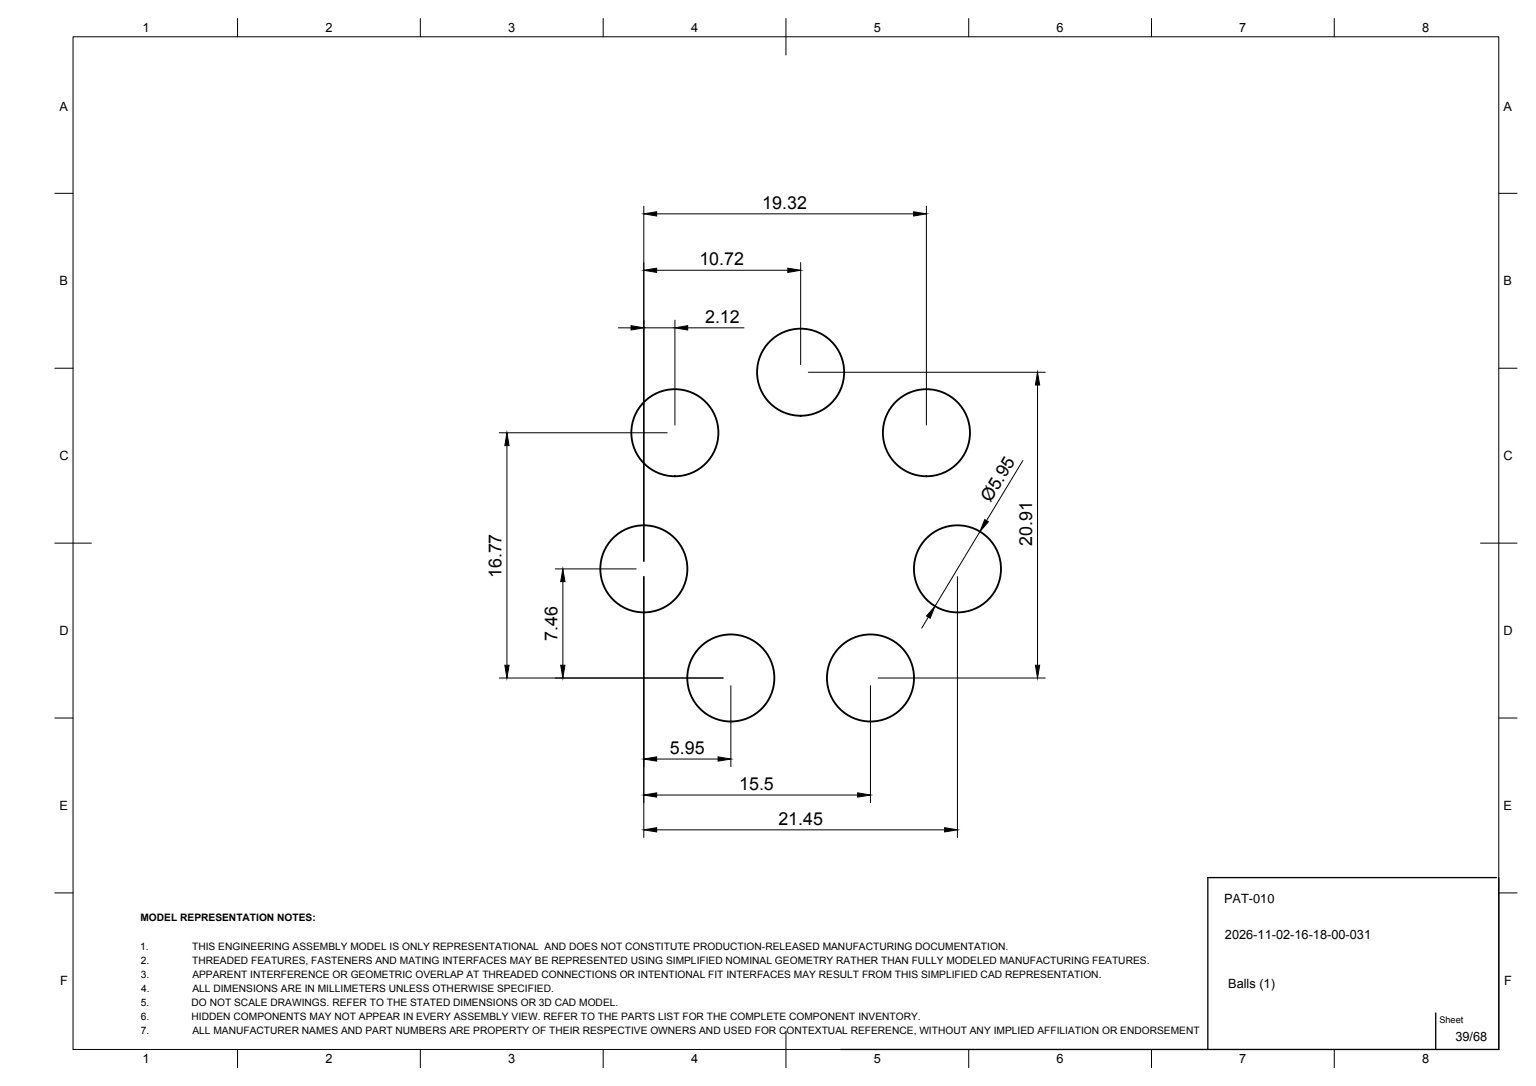
ISO-10303-21;
HEADER;
/* Generated by software containing ST-Developer
 * from STEP Tools, Inc. (www.steptools.com) 
 */

FILE_DESCRIPTION(
/* description */ ('Belt conveyor head drive unit'),
/* implementation_level */ '2;1');

FILE_NAME(
/* name */ 'Balls (1).step',
/* time_stamp */ '2026-10-28T03:26:19-07:00',
/* author */ (''),
/* organization */ (''),
/* preprocessor_version */ 'ST-DEVELOPER v20.2',
/* originating_system */ 'Autodesk Translation Framework v15.17.0.0',
/* authorisation */ '');

FILE_SCHEMA (('AUTOMOTIVE_DESIGN { 1 0 10303 214 3 1 1 }'));
ENDSEC;

DATA;
#10=MECHANICAL_DESIGN_GEOMETRIC_PRESENTATION_REPRESENTATION('',(#890,#891,#892,#893,#894,#895,#896),#27069);
#661=SPHERICAL_SURFACE('',#15395,0.29765);
#662=SPHERICAL_SURFACE('',#15397,0.29765);
#663=SPHERICAL_SURFACE('',#15399,0.29765);
#664=SPHERICAL_SURFACE('',#15401,0.29765);
#665=SPHERICAL_SURFACE('',#15403,0.29765);
#666=SPHERICAL_SURFACE('',#15405,0.29765);
#667=SPHERICAL_SURFACE('',#15407,0.29765);
#744=SHAPE_REPRESENTATION_RELATIONSHIP('SRR','None',#27390,#813);
#813=ADVANCED_BREP_SHAPE_REPRESENTATION('',(#974,#975,#976,#977,#978,#979,
#980),#27032);
#890=STYLED_ITEM('',(#27797),#974);
#891=STYLED_ITEM('',(#27797),#975);
#892=STYLED_ITEM('',(#27797),#976);
#893=STYLED_ITEM('',(#27797),#977);
#894=STYLED_ITEM('',(#27797),#978);
#895=STYLED_ITEM('',(#27797),#979);
#896=STYLED_ITEM('',(#27797),#980);
#974=MANIFOLD_SOLID_BREP('Body1',#13756);
#975=MANIFOLD_SOLID_BREP('Body2',#13757);
#976=MANIFOLD_SOLID_BREP('Body3',#13758);
#977=MANIFOLD_SOLID_BREP('Body4',#13759);
#978=MANIFOLD_SOLID_BREP('Body5',#13760);
#979=MANIFOLD_SOLID_BREP('Body6',#13761);
#980=MANIFOLD_SOLID_BREP('Body7',#13762);
#2021=FACE_OUTER_BOUND('',#2975,.T.);
#2022=FACE_OUTER_BOUND('',#2976,.T.);
#2023=FACE_OUTER_BOUND('',#2977,.T.);
#2024=FACE_OUTER_BOUND('',#2978,.T.);
#2025=FACE_OUTER_BOUND('',#2979,.T.);
#2026=FACE_OUTER_BOUND('',#2980,.T.);
#2027=FACE_OUTER_BOUND('',#2981,.T.);
#2975=EDGE_LOOP('',(#10618,#10619));
#2976=EDGE_LOOP('',(#10620,#10621));
#2977=EDGE_LOOP('',(#10622,#10623));
#2978=EDGE_LOOP('',(#10624,#10625));
#2979=EDGE_LOOP('',(#10626,#10627));
#2980=EDGE_LOOP('',(#10628,#10629));
#2981=EDGE_LOOP('',(#10630,#10631));
#5482=CIRCLE('',#15396,0.29765);
#5483=CIRCLE('',#15398,0.29765);
#5484=CIRCLE('',#15400,0.29765);
#5485=CIRCLE('',#15402,0.29765);
#5486=CIRCLE('',#15404,0.29765);
#5487=CIRCLE('',#15406,0.29765);
#5488=CIRCLE('',#15408,0.29765);
#6513=VERTEX_POINT('',#23132);
#6514=VERTEX_POINT('',#23133);
#6515=VERTEX_POINT('',#23136);
#6516=VERTEX_POINT('',#23137);
#6517=VERTEX_POINT('',#23140);
#6518=VERTEX_POINT('',#23141);
#6519=VERTEX_POINT('',#23144);
#6520=VERTEX_POINT('',#23145);
#6521=VERTEX_POINT('',#23148);
#6522=VERTEX_POINT('',#23149);
#6523=VERTEX_POINT('',#23152);
#6524=VERTEX_POINT('',#23153);
#6525=VERTEX_POINT('',#23156);
#6526=VERTEX_POINT('',#23157);
#8001=EDGE_CURVE('',#6513,#6514,#5482,.T.);
#8002=EDGE_CURVE('',#6515,#6516,#5483,.T.);
#8003=EDGE_CURVE('',#6517,#6518,#5484,.T.);
#8004=EDGE_CURVE('',#6519,#6520,#5485,.T.);
#8005=EDGE_CURVE('',#6521,#6522,#5486,.T.);
#8006=EDGE_CURVE('',#6523,#6524,#5487,.T.);
#8007=EDGE_CURVE('',#6525,#6526,#5488,.T.);
#10618=ORIENTED_EDGE('',*,*,#8001,.T.);
#10619=ORIENTED_EDGE('',*,*,#8001,.F.);
#10620=ORIENTED_EDGE('',*,*,#8002,.T.);
#10621=ORIENTED_EDGE('',*,*,#8002,.F.);
#10622=ORIENTED_EDGE('',*,*,#8003,.T.);
#10623=ORIENTED_EDGE('',*,*,#8003,.F.);
#10624=ORIENTED_EDGE('',*,*,#8004,.T.);
#10625=ORIENTED_EDGE('',*,*,#8004,.F.);
#10626=ORIENTED_EDGE('',*,*,#8005,.T.);
#10627=ORIENTED_EDGE('',*,*,#8005,.F.);
#10628=ORIENTED_EDGE('',*,*,#8006,.T.);
#10629=ORIENTED_EDGE('',*,*,#8006,.F.);
#10630=ORIENTED_EDGE('',*,*,#8007,.T.);
#10631=ORIENTED_EDGE('',*,*,#8007,.F.);
#13300=ADVANCED_FACE('',(#2021),#661,.T.);
#13301=ADVANCED_FACE('',(#2022),#662,.T.);
#13302=ADVANCED_FACE('',(#2023),#663,.T.);
#13303=ADVANCED_FACE('',(#2024),#664,.T.);
#13304=ADVANCED_FACE('',(#2025),#665,.T.);
#13305=ADVANCED_FACE('',(#2026),#666,.T.);
#13306=ADVANCED_FACE('',(#2027),#667,.T.);
#13756=CLOSED_SHELL('',(#13300));
#13757=CLOSED_SHELL('',(#13301));
#13758=CLOSED_SHELL('',(#13302));
#13759=CLOSED_SHELL('',(#13303));
#13760=CLOSED_SHELL('',(#13304));
#13761=CLOSED_SHELL('',(#13305));
#13762=CLOSED_SHELL('',(#13306));
#15394=AXIS2_PLACEMENT_3D('',#23130,#18510,#18511);
#15395=AXIS2_PLACEMENT_3D('',#23131,#18512,#18513);
#15396=AXIS2_PLACEMENT_3D('',#23134,#18514,#18515);
#15397=AXIS2_PLACEMENT_3D('',#23135,#18516,#18517);
#15398=AXIS2_PLACEMENT_3D('',#23138,#18518,#18519);
#15399=AXIS2_PLACEMENT_3D('',#23139,#18520,#18521);
#15400=AXIS2_PLACEMENT_3D('',#23142,#18522,#18523);
#15401=AXIS2_PLACEMENT_3D('',#23143,#18524,#18525);
#15402=AXIS2_PLACEMENT_3D('',#23146,#18526,#18527);
#15403=AXIS2_PLACEMENT_3D('',#23147,#18528,#18529);
#15404=AXIS2_PLACEMENT_3D('',#23150,#18530,#18531);
#15405=AXIS2_PLACEMENT_3D('',#23151,#18532,#18533);
#15406=AXIS2_PLACEMENT_3D('',#23154,#18534,#18535);
#15407=AXIS2_PLACEMENT_3D('',#23155,#18536,#18537);
#15408=AXIS2_PLACEMENT_3D('',#23158,#18538,#18539);
#18510=DIRECTION('axis',(0.,0.,1.));
#18511=DIRECTION('refdir',(1.,0.,0.));
#18512=DIRECTION('center_axis',(0.,0.,1.));
#18513=DIRECTION('ref_axis',(1.,0.,0.));
#18514=DIRECTION('center_axis',(1.22464679914735E-16,-1.,0.));
#18515=DIRECTION('ref_axis',(-1.,-1.22464679914735E-16,0.));
#18516=DIRECTION('center_axis',(0.78183148246803,0.,0.623489801858733));
#18517=DIRECTION('ref_axis',(0.623489801858734,0.,-0.78183148246803));
#18518=DIRECTION('center_axis',(7.63554790147315E-17,-1.,-9.57467422477103E-17));
#18519=DIRECTION('ref_axis',(-0.623489801858734,-1.22464679914735E-16,0.78183148246803));
#18520=DIRECTION('center_axis',(0.974927912181824,0.,-0.222520933956314));
#18521=DIRECTION('ref_axis',(-0.222520933956314,0.,-0.974927912181824));
#18522=DIRECTION('center_axis',(-2.7250954951288E-17,-1.,-1.19394234705288E-16));
#18523=DIRECTION('ref_axis',(0.222520933956314,-1.22464679914735E-16,0.974927912181824));
#18524=DIRECTION('center_axis',(0.433883739117558,0.,-0.900968867902419));
#18525=DIRECTION('ref_axis',(-0.900968867902419,0.,-0.433883739117558));
#18526=DIRECTION('center_axis',(-1.10336864020811E-16,-1.,-5.31354332312403E-17));
#18527=DIRECTION('ref_axis',(0.900968867902419,-1.22464679914735E-16,0.433883739117558));
#18528=DIRECTION('center_axis',(-0.433883739117558,0.,-0.900968867902419));
#18529=DIRECTION('ref_axis',(-0.900968867902419,0.,0.433883739117558));
#18530=DIRECTION('center_axis',(-1.10336864020811E-16,-1.,5.31354332312403E-17));
#18531=DIRECTION('ref_axis',(0.900968867902419,-1.22464679914735E-16,-0.433883739117558));
#18532=DIRECTION('center_axis',(-0.974927912181824,0.,-0.222520933956314));
#18533=DIRECTION('ref_axis',(-0.222520933956315,0.,0.974927912181824));
#18534=DIRECTION('center_axis',(-2.7250954951288E-17,-1.,1.19394234705288E-16));
#18535=DIRECTION('ref_axis',(0.222520933956315,-1.22464679914735E-16,-0.974927912181824));
#18536=DIRECTION('center_axis',(-0.78183148246803,0.,0.623489801858734));
#18537=DIRECTION('ref_axis',(0.623489801858733,0.,0.78183148246803));
#18538=DIRECTION('center_axis',(7.63554790147315E-17,-1.,9.57467422477103E-17));
#18539=DIRECTION('ref_axis',(-0.623489801858733,-1.22464679914735E-16,-0.78183148246803));
#23130=CARTESIAN_POINT('',(0.,0.,0.));
#23131=CARTESIAN_POINT('Origin',(1.1,0.,0.));
#23132=CARTESIAN_POINT('',(1.1,-2.23201749654651E-33,0.29765));
#23133=CARTESIAN_POINT('',(1.1,-2.23201749654651E-33,-0.29765));
#23134=CARTESIAN_POINT('Origin',(1.1,0.,0.));
#23135=CARTESIAN_POINT('Origin',(0.685838782044607,0.,-0.860014630714833));
#23136=CARTESIAN_POINT('',(0.918550922801216,-5.31350540756609E-33,-0.674432891191581));
#23137=CARTESIAN_POINT('',(0.453126641287998,8.49470414473068E-34,-1.04559637023808));
#23138=CARTESIAN_POINT('Origin',(0.685838782044607,0.,-0.860014630714833));
#23139=CARTESIAN_POINT('Origin',(-0.244773027351946,0.,-1.07242070340001));
#23140=CARTESIAN_POINT('',(0.0454142657089739,-2.23201749654651E-33,-1.1386540593921));
#23141=CARTESIAN_POINT('',(-0.534960320412865,-2.23201749654651E-33,-1.00618734740791));
#23142=CARTESIAN_POINT('Origin',(-0.244773027351946,0.,-1.07242070340001));
#23143=CARTESIAN_POINT('Origin',(-0.991065754692661,0.,-0.477272113029314));
#23144=CARTESIAN_POINT('',(-0.86192025974432,8.49470414473067E-34,-0.745445496560469));
#23145=CARTESIAN_POINT('',(-1.120211249641,-5.31350540756609E-33,-0.209098729498159));
#23146=CARTESIAN_POINT('Origin',(-0.991065754692661,0.,-0.477272113029314));
#23147=CARTESIAN_POINT('Origin',(-0.991065754692661,0.,0.477272113029314));
#23148=CARTESIAN_POINT('',(-1.120211249641,-2.23201749654651E-33,0.209098729498159));
#23149=CARTESIAN_POINT('',(-0.86192025974432,-2.23201749654651E-33,0.745445496560469));
#23150=CARTESIAN_POINT('Origin',(-0.991065754692661,0.,0.477272113029314));
#23151=CARTESIAN_POINT('Origin',(-0.244773027351946,0.,1.07242070340001));
#23152=CARTESIAN_POINT('',(-0.534960320412866,-2.23201749654651E-33,1.00618734740791));
#23153=CARTESIAN_POINT('',(0.0454142657089737,-2.23201749654651E-33,1.1386540593921));
#23154=CARTESIAN_POINT('Origin',(-0.244773027351946,0.,1.07242070340001));
#23155=CARTESIAN_POINT('Origin',(0.685838782044607,0.,0.860014630714833));
#23156=CARTESIAN_POINT('',(0.453126641287998,-2.23201749654651E-33,1.04559637023808));
#23157=CARTESIAN_POINT('',(0.918550922801216,-2.23201749654651E-33,0.674432891191581));
#23158=CARTESIAN_POINT('Origin',(0.685838782044607,0.,0.860014630714833));
#26955=UNCERTAINTY_MEASURE_WITH_UNIT(LENGTH_MEASURE(0.001),#27070,
'DISTANCE_ACCURACY_VALUE',
'Maximum model space distance between geometric entities at asserted c
onnectivities');
#26992=UNCERTAINTY_MEASURE_WITH_UNIT(LENGTH_MEASURE(0.001),#27070,
'DISTANCE_ACCURACY_VALUE',
'Maximum model space distance between geometric entities at asserted c
onnectivities');
#27032=(
GEOMETRIC_REPRESENTATION_CONTEXT(3)
GLOBAL_UNCERTAINTY_ASSIGNED_CONTEXT((#26955))
GLOBAL_UNIT_ASSIGNED_CONTEXT((#27070,#27072,#27073))
REPRESENTATION_CONTEXT('','3D')
);
#27069=(
GEOMETRIC_REPRESENTATION_CONTEXT(3)
GLOBAL_UNCERTAINTY_ASSIGNED_CONTEXT((#26992))
GLOBAL_UNIT_ASSIGNED_CONTEXT((#27070,#27072,#27073))
REPRESENTATION_CONTEXT('','3D')
);
#27070=(
LENGTH_UNIT()
NAMED_UNIT(*)
SI_UNIT(.CENTI.,.METRE.)
);
#27072=(
NAMED_UNIT(*)
PLANE_ANGLE_UNIT()
SI_UNIT($,.RADIAN.)
);
#27073=(
NAMED_UNIT(*)
SI_UNIT($,.STERADIAN.)
SOLID_ANGLE_UNIT()
);
#27113=SHAPE_DEFINITION_REPRESENTATION(#27194,#27390);
#27194=PRODUCT_DEFINITION_SHAPE('',$,#27467);
#27390=SHAPE_REPRESENTATION('',(#15394),#27032);
#27427=PRODUCT_DEFINITION_CONTEXT('part definition',#27657,'design');
#27467=PRODUCT_DEFINITION('Balls (1)','Balls (1)',#27543,#27427);
#27543=PRODUCT_DEFINITION_FORMATION('',$,#27698);
#27657=APPLICATION_CONTEXT(
'Core Data for Automotive Mechanical Design Process');
#27658=PRODUCT_CONTEXT('part definition',#27657,'mechanical');
#27698=PRODUCT('Balls (1)','Balls (1)','Balls (1)',(#27658));
#27791=COLOUR_RGB('Grey',0.48,0.52,0.57);
#27792=FILL_AREA_STYLE_COLOUR('',#27791);
#27793=FILL_AREA_STYLE('',(#27792));
#27794=SURFACE_STYLE_FILL_AREA(#27793);
#27795=SURFACE_SIDE_STYLE('',(#27794));
#27796=SURFACE_STYLE_USAGE(.BOTH.,#27795);
#27797=PRESENTATION_STYLE_ASSIGNMENT((#27796));
ENDSEC;
END-ISO-10303-21;
